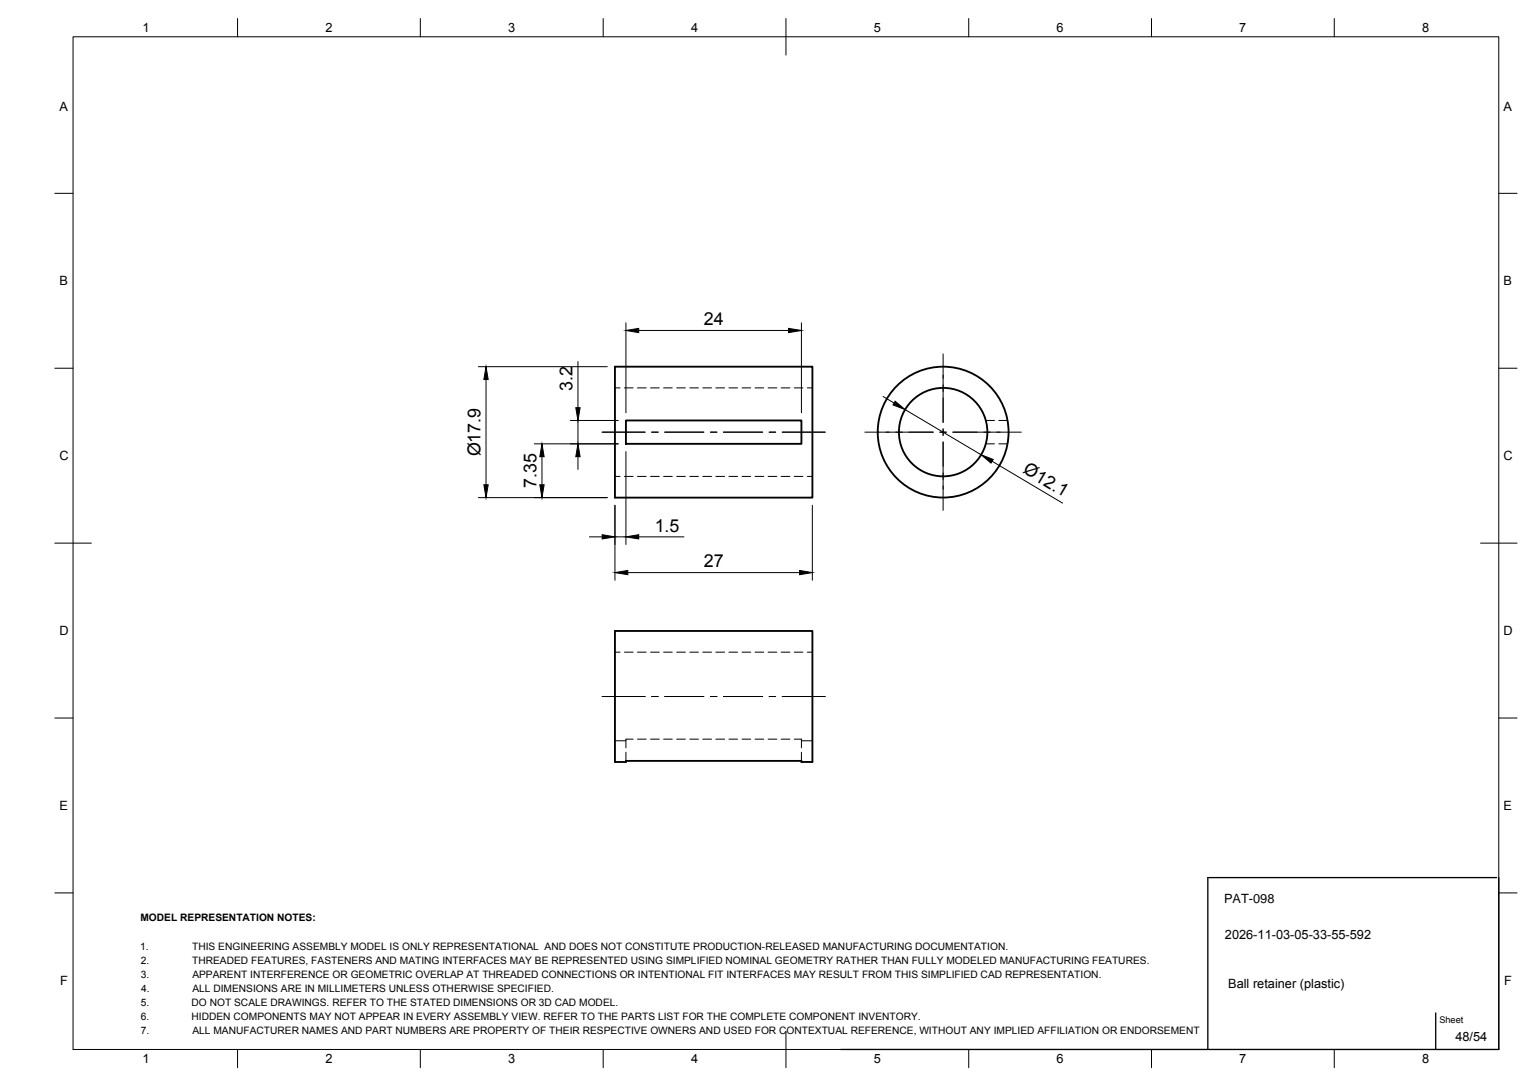
ISO-10303-21;
HEADER;
/* Generated by software containing ST-Developer
 * from STEP Tools, Inc. (www.steptools.com) 
 */

FILE_DESCRIPTION(
/* description */ ('Spring compression tester'),
/* implementation_level */ '2;1');

FILE_NAME(
/* name */ 'Ball retainer (plastic).step',
/* time_stamp */ '2026-10-28T03:24:11-07:00',
/* author */ (''),
/* organization */ (''),
/* preprocessor_version */ 'ST-DEVELOPER v20.2',
/* originating_system */ 'Autodesk Translation Framework v15.17.0.0',
/* authorisation */ '');

FILE_SCHEMA (('AUTOMOTIVE_DESIGN { 1 0 10303 214 3 1 1 }'));
ENDSEC;

DATA;
#10=MECHANICAL_DESIGN_GEOMETRIC_PRESENTATION_REPRESENTATION('',(#1165),#43521);
#1030=SHAPE_REPRESENTATION_RELATIONSHIP('SRR','None',#43846,#1090);
#1090=ADVANCED_BREP_SHAPE_REPRESENTATION('',(#1236),#43506);
#1165=STYLED_ITEM('',(#44195),#1236);
#1236=MANIFOLD_SOLID_BREP('Body1',#18606);
#1549=FACE_BOUND('',#4279,.T.);
#1550=FACE_BOUND('',#4281,.T.);
#1551=FACE_BOUND('',#4283,.T.);
#1552=FACE_BOUND('',#4285,.T.);
#2077=PLANE('',#20673);
#2078=PLANE('',#20676);
#2079=PLANE('',#20677);
#2080=PLANE('',#20680);
#2081=PLANE('',#20681);
#2082=PLANE('',#20686);
#2925=FACE_OUTER_BOUND('',#4274,.T.);
#2926=FACE_OUTER_BOUND('',#4275,.T.);
#2927=FACE_OUTER_BOUND('',#4276,.T.);
#2928=FACE_OUTER_BOUND('',#4277,.T.);
#2929=FACE_OUTER_BOUND('',#4278,.T.);
#2930=FACE_OUTER_BOUND('',#4280,.T.);
#2931=FACE_OUTER_BOUND('',#4282,.T.);
#2932=FACE_OUTER_BOUND('',#4284,.T.);
#4274=EDGE_LOOP('',(#15639,#15640,#15641,#15642));
#4275=EDGE_LOOP('',(#15643,#15644,#15645,#15646));
#4276=EDGE_LOOP('',(#15647,#15648,#15649,#15650));
#4277=EDGE_LOOP('',(#15651,#15652,#15653,#15654));
#4278=EDGE_LOOP('',(#15655));
#4279=EDGE_LOOP('',(#15656));
#4280=EDGE_LOOP('',(#15657,#15658,#15659,#15660));
#4281=EDGE_LOOP('',(#15661,#15662,#15663,#15664));
#4282=EDGE_LOOP('',(#15665));
#4283=EDGE_LOOP('',(#15666));
#4284=EDGE_LOOP('',(#15667,#15668,#15669,#15670));
#4285=EDGE_LOOP('',(#15671,#15672,#15673,#15674));
#5714=LINE('',#30770,#7146);
#5715=LINE('',#30773,#7147);
#5716=LINE('',#30776,#7148);
#5717=LINE('',#30778,#7149);
#5718=LINE('',#30779,#7150);
#5719=LINE('',#30785,#7151);
#5720=LINE('',#30787,#7152);
#5721=LINE('',#30788,#7153);
#5722=LINE('',#30797,#7154);
#5723=LINE('',#30802,#7155);
#7146=VECTOR('',#25086,1.);
#7147=VECTOR('',#25089,1.);
#7148=VECTOR('',#25092,1.);
#7149=VECTOR('',#25093,1.);
#7150=VECTOR('',#25094,1.);
#7151=VECTOR('',#25101,1.);
#7152=VECTOR('',#25104,1.);
#7153=VECTOR('',#25105,1.);
#7154=VECTOR('',#25116,0.895);
#7155=VECTOR('',#25123,0.605);
#8039=CIRCLE('',#20674,0.895);
#8040=CIRCLE('',#20675,0.605);
#8041=CIRCLE('',#20678,0.895);
#8042=CIRCLE('',#20679,0.605);
#8043=CIRCLE('',#20682,0.895);
#8044=CIRCLE('',#20683,0.605);
#8045=CIRCLE('',#20685,0.895);
#8046=CIRCLE('',#20687,0.605);
#9288=VERTEX_POINT('',#30766);
#9289=VERTEX_POINT('',#30767);
#9290=VERTEX_POINT('',#30769);
#9291=VERTEX_POINT('',#30771);
#9292=VERTEX_POINT('',#30775);
#9293=VERTEX_POINT('',#30777);
#9294=VERTEX_POINT('',#30781);
#9295=VERTEX_POINT('',#30783);
#9296=VERTEX_POINT('',#30790);
#9297=VERTEX_POINT('',#30792);
#9298=VERTEX_POINT('',#30795);
#9299=VERTEX_POINT('',#30799);
#11484=EDGE_CURVE('',#9288,#9289,#8039,.T.);
#11485=EDGE_CURVE('',#9290,#9288,#5714,.T.);
#11486=EDGE_CURVE('',#9291,#9290,#8040,.T.);
#11487=EDGE_CURVE('',#9289,#9291,#5715,.T.);
#11488=EDGE_CURVE('',#9289,#9292,#5716,.T.);
#11489=EDGE_CURVE('',#9293,#9291,#5717,.T.);
#11490=EDGE_CURVE('',#9293,#9292,#5718,.T.);
#11491=EDGE_CURVE('',#9292,#9294,#8041,.T.);
#11492=EDGE_CURVE('',#9295,#9293,#8042,.T.);
#11493=EDGE_CURVE('',#9294,#9295,#5719,.T.);
#11494=EDGE_CURVE('',#9294,#9288,#5720,.T.);
#11495=EDGE_CURVE('',#9290,#9295,#5721,.T.);
#11496=EDGE_CURVE('',#9296,#9296,#8043,.T.);
#11497=EDGE_CURVE('',#9297,#9297,#8044,.T.);
#11498=EDGE_CURVE('',#9298,#9298,#8045,.T.);
#11499=EDGE_CURVE('',#9298,#9296,#5722,.T.);
#11500=EDGE_CURVE('',#9299,#9299,#8046,.T.);
#11501=EDGE_CURVE('',#9299,#9297,#5723,.T.);
#15639=ORIENTED_EDGE('',*,*,#11484,.F.);
#15640=ORIENTED_EDGE('',*,*,#11485,.F.);
#15641=ORIENTED_EDGE('',*,*,#11486,.F.);
#15642=ORIENTED_EDGE('',*,*,#11487,.F.);
#15643=ORIENTED_EDGE('',*,*,#11488,.F.);
#15644=ORIENTED_EDGE('',*,*,#11487,.T.);
#15645=ORIENTED_EDGE('',*,*,#11489,.F.);
#15646=ORIENTED_EDGE('',*,*,#11490,.T.);
#15647=ORIENTED_EDGE('',*,*,#11491,.F.);
#15648=ORIENTED_EDGE('',*,*,#11490,.F.);
#15649=ORIENTED_EDGE('',*,*,#11492,.F.);
#15650=ORIENTED_EDGE('',*,*,#11493,.F.);
#15651=ORIENTED_EDGE('',*,*,#11494,.F.);
#15652=ORIENTED_EDGE('',*,*,#11493,.T.);
#15653=ORIENTED_EDGE('',*,*,#11495,.F.);
#15654=ORIENTED_EDGE('',*,*,#11485,.T.);
#15655=ORIENTED_EDGE('',*,*,#11496,.F.);
#15656=ORIENTED_EDGE('',*,*,#11497,.T.);
#15657=ORIENTED_EDGE('',*,*,#11498,.F.);
#15658=ORIENTED_EDGE('',*,*,#11499,.T.);
#15659=ORIENTED_EDGE('',*,*,#11496,.T.);
#15660=ORIENTED_EDGE('',*,*,#11499,.F.);
#15661=ORIENTED_EDGE('',*,*,#11491,.T.);
#15662=ORIENTED_EDGE('',*,*,#11494,.T.);
#15663=ORIENTED_EDGE('',*,*,#11484,.T.);
#15664=ORIENTED_EDGE('',*,*,#11488,.T.);
#15665=ORIENTED_EDGE('',*,*,#11498,.T.);
#15666=ORIENTED_EDGE('',*,*,#11500,.F.);
#15667=ORIENTED_EDGE('',*,*,#11500,.T.);
#15668=ORIENTED_EDGE('',*,*,#11501,.T.);
#15669=ORIENTED_EDGE('',*,*,#11497,.F.);
#15670=ORIENTED_EDGE('',*,*,#11501,.F.);
#15671=ORIENTED_EDGE('',*,*,#11492,.T.);
#15672=ORIENTED_EDGE('',*,*,#11489,.T.);
#15673=ORIENTED_EDGE('',*,*,#11486,.T.);
#15674=ORIENTED_EDGE('',*,*,#11495,.T.);
#17312=CYLINDRICAL_SURFACE('',#20684,0.895);
#17313=CYLINDRICAL_SURFACE('',#20688,0.605);
#18249=ADVANCED_FACE('',(#2925),#2077,.F.);
#18250=ADVANCED_FACE('',(#2926),#2078,.F.);
#18251=ADVANCED_FACE('',(#2927),#2079,.F.);
#18252=ADVANCED_FACE('',(#2928),#2080,.F.);
#18253=ADVANCED_FACE('',(#2929,#1549),#2081,.T.);
#18254=ADVANCED_FACE('',(#2930,#1550),#17312,.T.);
#18255=ADVANCED_FACE('',(#2931,#1551),#2082,.T.);
#18256=ADVANCED_FACE('',(#2932,#1552),#17313,.F.);
#18606=CLOSED_SHELL('',(#18249,#18250,#18251,#18252,#18253,#18254,#18255,
#18256));
#20672=AXIS2_PLACEMENT_3D('',#30764,#25080,#25081);
#20673=AXIS2_PLACEMENT_3D('',#30765,#25082,#25083);
#20674=AXIS2_PLACEMENT_3D('',#30768,#25084,#25085);
#20675=AXIS2_PLACEMENT_3D('',#30772,#25087,#25088);
#20676=AXIS2_PLACEMENT_3D('',#30774,#25090,#25091);
#20677=AXIS2_PLACEMENT_3D('',#30780,#25095,#25096);
#20678=AXIS2_PLACEMENT_3D('',#30782,#25097,#25098);
#20679=AXIS2_PLACEMENT_3D('',#30784,#25099,#25100);
#20680=AXIS2_PLACEMENT_3D('',#30786,#25102,#25103);
#20681=AXIS2_PLACEMENT_3D('',#30789,#25106,#25107);
#20682=AXIS2_PLACEMENT_3D('',#30791,#25108,#25109);
#20683=AXIS2_PLACEMENT_3D('',#30793,#25110,#25111);
#20684=AXIS2_PLACEMENT_3D('',#30794,#25112,#25113);
#20685=AXIS2_PLACEMENT_3D('',#30796,#25114,#25115);
#20686=AXIS2_PLACEMENT_3D('',#30798,#25117,#25118);
#20687=AXIS2_PLACEMENT_3D('',#30800,#25119,#25120);
#20688=AXIS2_PLACEMENT_3D('',#30801,#25121,#25122);
#25080=DIRECTION('axis',(0.,0.,1.));
#25081=DIRECTION('refdir',(1.,0.,0.));
#25082=DIRECTION('center_axis',(0.,1.,0.));
#25083=DIRECTION('ref_axis',(0.,0.,1.));
#25084=DIRECTION('center_axis',(0.,1.,0.));
#25085=DIRECTION('ref_axis',(1.,0.,0.));
#25086=DIRECTION('',(1.,0.,0.));
#25087=DIRECTION('center_axis',(0.,-1.,0.));
#25088=DIRECTION('ref_axis',(1.,0.,0.));
#25089=DIRECTION('',(-1.,0.,0.));
#25090=DIRECTION('center_axis',(0.,0.,-1.));
#25091=DIRECTION('ref_axis',(-1.,0.,0.));
#25092=DIRECTION('',(0.,-1.,0.));
#25093=DIRECTION('',(0.,1.,0.));
#25094=DIRECTION('',(1.,0.,0.));
#25095=DIRECTION('center_axis',(0.,-1.,0.));
#25096=DIRECTION('ref_axis',(0.,0.,-1.));
#25097=DIRECTION('center_axis',(0.,-1.,0.));
#25098=DIRECTION('ref_axis',(1.,0.,0.));
#25099=DIRECTION('center_axis',(0.,1.,0.));
#25100=DIRECTION('ref_axis',(1.,0.,0.));
#25101=DIRECTION('',(-1.,0.,0.));
#25102=DIRECTION('center_axis',(0.,0.,1.));
#25103=DIRECTION('ref_axis',(1.,0.,0.));
#25104=DIRECTION('',(0.,1.,0.));
#25105=DIRECTION('',(0.,-1.,0.));
#25106=DIRECTION('center_axis',(0.,1.,0.));
#25107=DIRECTION('ref_axis',(0.,0.,1.));
#25108=DIRECTION('center_axis',(0.,-1.,0.));
#25109=DIRECTION('ref_axis',(1.,0.,0.));
#25110=DIRECTION('center_axis',(0.,-1.,0.));
#25111=DIRECTION('ref_axis',(1.,0.,0.));
#25112=DIRECTION('center_axis',(0.,-1.,0.));
#25113=DIRECTION('ref_axis',(1.,0.,0.));
#25114=DIRECTION('center_axis',(0.,-1.,0.));
#25115=DIRECTION('ref_axis',(1.,0.,0.));
#25116=DIRECTION('',(0.,1.,0.));
#25117=DIRECTION('center_axis',(0.,-1.,0.));
#25118=DIRECTION('ref_axis',(0.,0.,-1.));
#25119=DIRECTION('center_axis',(0.,-1.,0.));
#25120=DIRECTION('ref_axis',(1.,0.,0.));
#25121=DIRECTION('center_axis',(0.,-1.,0.));
#25122=DIRECTION('ref_axis',(1.,0.,0.));
#25123=DIRECTION('',(0.,1.,0.));
#30764=CARTESIAN_POINT('',(0.,0.,0.));
#30765=CARTESIAN_POINT('Origin',(0.75,1.2,0.));
#30766=CARTESIAN_POINT('',(0.880582193778639,1.2,0.16));
#30767=CARTESIAN_POINT('',(0.880582193778639,1.2,-0.16));
#30768=CARTESIAN_POINT('Origin',(0.,1.2,0.));
#30769=CARTESIAN_POINT('',(0.583459510163302,1.2,0.16));
#30770=CARTESIAN_POINT('',(0.57,1.2,0.16));
#30771=CARTESIAN_POINT('',(0.583459510163302,1.2,-0.16));
#30772=CARTESIAN_POINT('Origin',(0.,1.2,0.));
#30773=CARTESIAN_POINT('',(0.93,1.2,-0.16));
#30774=CARTESIAN_POINT('Origin',(0.93,0.,-0.16));
#30775=CARTESIAN_POINT('',(0.880582193778639,-1.2,-0.16));
#30776=CARTESIAN_POINT('',(0.880582193778639,0.,-0.16));
#30777=CARTESIAN_POINT('',(0.583459510163302,-1.2,-0.16));
#30778=CARTESIAN_POINT('',(0.583459510163302,0.,-0.16));
#30779=CARTESIAN_POINT('',(0.93,-1.2,-0.16));
#30780=CARTESIAN_POINT('Origin',(0.75,-1.2,0.));
#30781=CARTESIAN_POINT('',(0.880582193778639,-1.2,0.16));
#30782=CARTESIAN_POINT('Origin',(0.,-1.2,0.));
#30783=CARTESIAN_POINT('',(0.583459510163302,-1.2,0.16));
#30784=CARTESIAN_POINT('Origin',(0.,-1.2,0.));
#30785=CARTESIAN_POINT('',(0.57,-1.2,0.16));
#30786=CARTESIAN_POINT('Origin',(0.57,0.,0.16));
#30787=CARTESIAN_POINT('',(0.880582193778639,0.,0.16));
#30788=CARTESIAN_POINT('',(0.583459510163302,0.,0.16));
#30789=CARTESIAN_POINT('Origin',(0.895,1.35,0.));
#30790=CARTESIAN_POINT('',(-0.895,1.35,-1.09605888523688E-16));
#30791=CARTESIAN_POINT('Origin',(0.,1.35,0.));
#30792=CARTESIAN_POINT('',(-0.605,1.35,-7.40911313484149E-17));
#30793=CARTESIAN_POINT('Origin',(0.,1.35,0.));
#30794=CARTESIAN_POINT('Origin',(0.,0.,0.));
#30795=CARTESIAN_POINT('',(-0.895,-1.35,-1.09605888523688E-16));
#30796=CARTESIAN_POINT('Origin',(0.,-1.35,0.));
#30797=CARTESIAN_POINT('',(-0.895,0.,-1.09605888523688E-16));
#30798=CARTESIAN_POINT('Origin',(0.605,-1.35,0.));
#30799=CARTESIAN_POINT('',(-0.605,-1.35,-7.40911313484149E-17));
#30800=CARTESIAN_POINT('Origin',(0.,-1.35,0.));
#30801=CARTESIAN_POINT('Origin',(0.,0.,0.));
#30802=CARTESIAN_POINT('',(-0.605,0.,-7.40911313484149E-17));
#43438=UNCERTAINTY_MEASURE_WITH_UNIT(LENGTH_MEASURE(0.001),#43522,
'DISTANCE_ACCURACY_VALUE',
'Maximum model space distance between geometric entities at asserted c
onnectivities');
#43453=UNCERTAINTY_MEASURE_WITH_UNIT(LENGTH_MEASURE(0.001),#43522,
'DISTANCE_ACCURACY_VALUE',
'Maximum model space distance between geometric entities at asserted c
onnectivities');
#43506=(
GEOMETRIC_REPRESENTATION_CONTEXT(3)
GLOBAL_UNCERTAINTY_ASSIGNED_CONTEXT((#43438))
GLOBAL_UNIT_ASSIGNED_CONTEXT((#43522,#43524,#43525))
REPRESENTATION_CONTEXT('','3D')
);
#43521=(
GEOMETRIC_REPRESENTATION_CONTEXT(3)
GLOBAL_UNCERTAINTY_ASSIGNED_CONTEXT((#43453))
GLOBAL_UNIT_ASSIGNED_CONTEXT((#43522,#43524,#43525))
REPRESENTATION_CONTEXT('','3D')
);
#43522=(
LENGTH_UNIT()
NAMED_UNIT(*)
SI_UNIT(.CENTI.,.METRE.)
);
#43524=(
NAMED_UNIT(*)
PLANE_ANGLE_UNIT()
SI_UNIT($,.RADIAN.)
);
#43525=(
NAMED_UNIT(*)
SI_UNIT($,.STERADIAN.)
SOLID_ANGLE_UNIT()
);
#43578=SHAPE_DEFINITION_REPRESENTATION(#43655,#43846);
#43655=PRODUCT_DEFINITION_SHAPE('',$,#43914);
#43846=SHAPE_REPRESENTATION('',(#20672),#43506);
#43861=PRODUCT_DEFINITION_CONTEXT('part definition',#44064,'design');
#43914=PRODUCT_DEFINITION('Ball retainer (plastic)',
'Ball retainer (plastic)',#43981,#43861);
#43981=PRODUCT_DEFINITION_FORMATION('',$,#44118);
#44064=APPLICATION_CONTEXT(
'Core Data for Automotive Mechanical Design Process');
#44065=PRODUCT_CONTEXT('part definition',#44064,'mechanical');
#44118=PRODUCT('Ball retainer (plastic)','Ball retainer (plastic)',
'Ball retainer (plastic)',(#44065));
#44189=COLOUR_RGB('Sky Blue',0.24,0.69,0.87);
#44190=FILL_AREA_STYLE_COLOUR('',#44189);
#44191=FILL_AREA_STYLE('',(#44190));
#44192=SURFACE_STYLE_FILL_AREA(#44191);
#44193=SURFACE_SIDE_STYLE('',(#44192));
#44194=SURFACE_STYLE_USAGE(.BOTH.,#44193);
#44195=PRESENTATION_STYLE_ASSIGNMENT((#44194));
ENDSEC;
END-ISO-10303-21;
